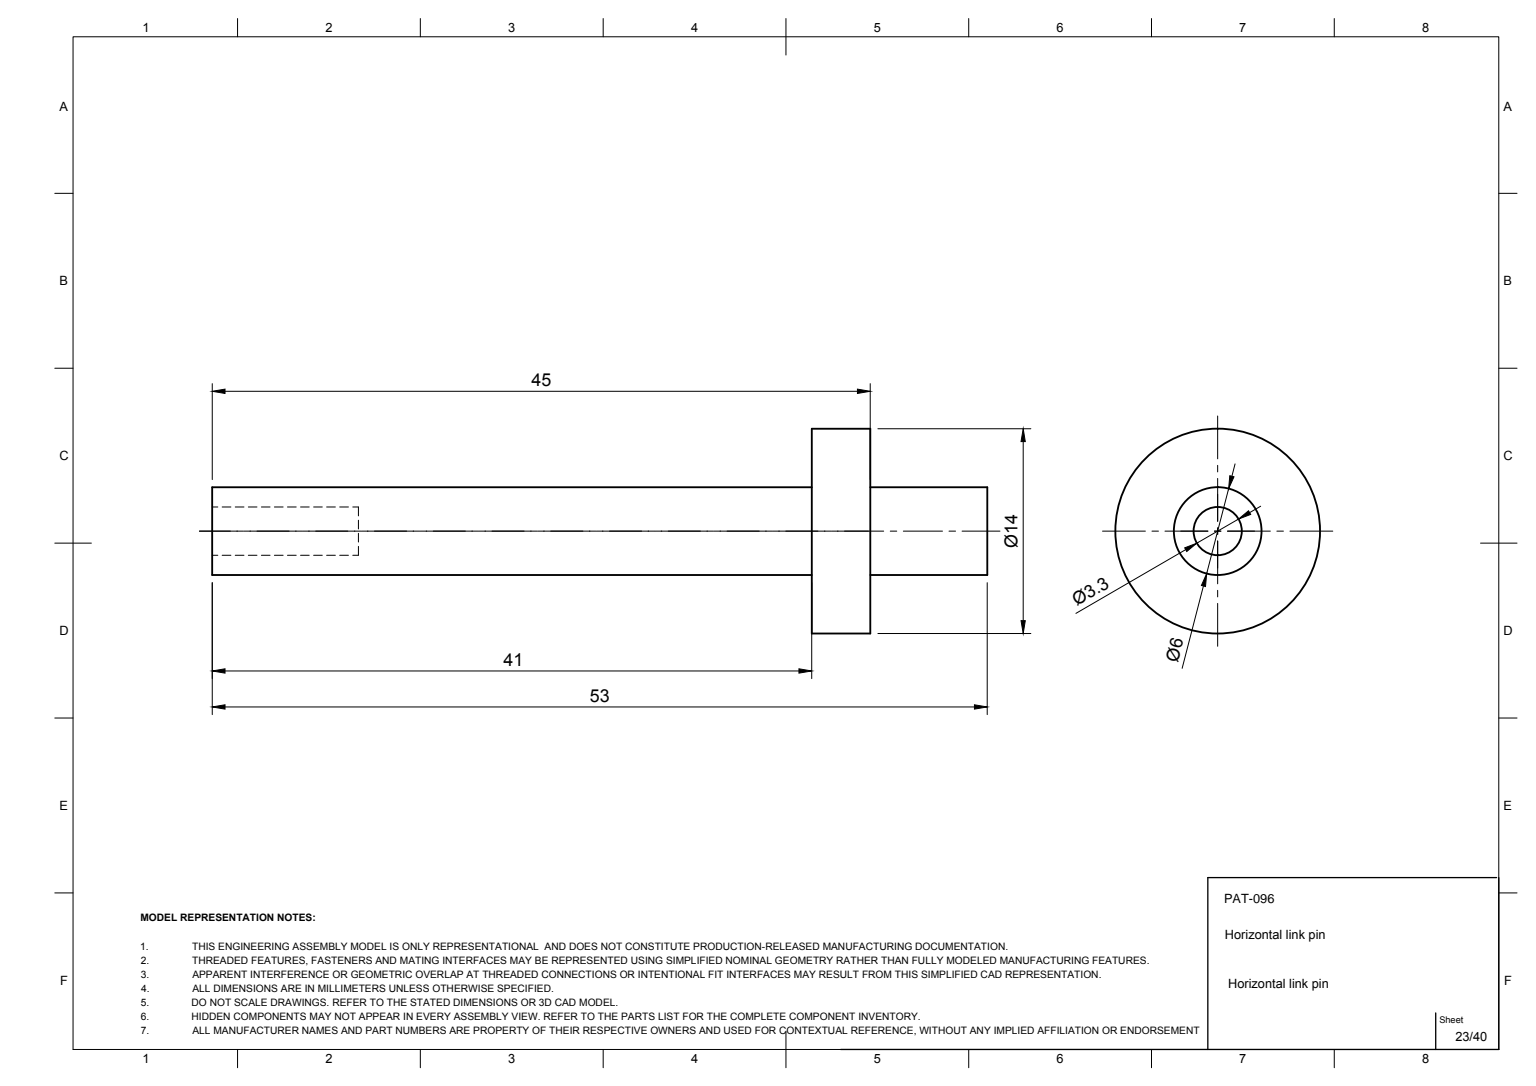
ISO-10303-21;
HEADER;
/* Generated by software containing ST-Developer
 * from STEP Tools, Inc. (www.steptools.com) 
 */

FILE_DESCRIPTION(
/* description */ ('PAT-096'),
/* implementation_level */ '2;1');

FILE_NAME(
/* name */ 'Horizontal link pin.step',
/* time_stamp */ '2026-10-29T17:03:14-07:00',
/* author */ (''),
/* organization */ (''),
/* preprocessor_version */ 'ST-DEVELOPER v20.2',
/* originating_system */ 'Autodesk Translation Framework v15.17.0.0',
/* authorisation */ '');

FILE_SCHEMA (('AUTOMOTIVE_DESIGN { 1 0 10303 214 3 1 1 }'));
ENDSEC;

DATA;
#10=MECHANICAL_DESIGN_GEOMETRIC_PRESENTATION_REPRESENTATION('',(#424),#10650);
#354=SHAPE_REPRESENTATION_RELATIONSHIP('SRR','None',#10816,#385);
#385=ADVANCED_BREP_SHAPE_REPRESENTATION('',(#461),#10634);
#424=STYLED_ITEM('',(#11064),#461);
#461=MANIFOLD_SOLID_BREP('Body1',#5559);
#559=FACE_BOUND('',#1440,.T.);
#560=FACE_BOUND('',#1442,.T.);
#561=FACE_BOUND('',#1447,.T.);
#725=PLANE('',#6395);
#726=PLANE('',#6396);
#727=PLANE('',#6399);
#728=PLANE('',#6407);
#729=PLANE('',#6408);
#1015=FACE_OUTER_BOUND('',#1437,.T.);
#1016=FACE_OUTER_BOUND('',#1438,.T.);
#1017=FACE_OUTER_BOUND('',#1439,.T.);
#1018=FACE_OUTER_BOUND('',#1441,.T.);
#1019=FACE_OUTER_BOUND('',#1443,.T.);
#1020=FACE_OUTER_BOUND('',#1444,.T.);
#1021=FACE_OUTER_BOUND('',#1445,.T.);
#1022=FACE_OUTER_BOUND('',#1446,.T.);
#1023=FACE_OUTER_BOUND('',#1448,.T.);
#1437=EDGE_LOOP('',(#4659,#4660,#4661,#4662));
#1438=EDGE_LOOP('',(#4663));
#1439=EDGE_LOOP('',(#4664));
#1440=EDGE_LOOP('',(#4665));
#1441=EDGE_LOOP('',(#4666));
#1442=EDGE_LOOP('',(#4667));
#1443=EDGE_LOOP('',(#4668,#4669,#4670,#4671));
#1444=EDGE_LOOP('',(#4672,#4673,#4674,#4675));
#1445=EDGE_LOOP('',(#4676,#4677,#4678,#4679));
#1446=EDGE_LOOP('',(#4680));
#1447=EDGE_LOOP('',(#4681));
#1448=EDGE_LOOP('',(#4682));
#1818=LINE('',#10049,#2147);
#1819=LINE('',#10063,#2148);
#1820=LINE('',#10066,#2149);
#1821=LINE('',#10071,#2150);
#2147=VECTOR('',#7846,0.165);
#2148=VECTOR('',#7865,0.7);
#2149=VECTOR('',#7868,0.3);
#2150=VECTOR('',#7875,0.3);
#2483=CIRCLE('',#6393,0.165);
#2484=CIRCLE('',#6394,0.165);
#2485=CIRCLE('',#6397,0.7);
#2486=CIRCLE('',#6398,0.3);
#2487=CIRCLE('',#6400,0.7);
#2488=CIRCLE('',#6401,0.3);
#2489=CIRCLE('',#6404,0.3);
#2490=CIRCLE('',#6406,0.3);
#2899=VERTEX_POINT('',#10046);
#2900=VERTEX_POINT('',#10048);
#2901=VERTEX_POINT('',#10053);
#2902=VERTEX_POINT('',#10055);
#2903=VERTEX_POINT('',#10058);
#2904=VERTEX_POINT('',#10060);
#2905=VERTEX_POINT('',#10065);
#2906=VERTEX_POINT('',#10069);
#3508=EDGE_CURVE('',#2899,#2899,#2483,.T.);
#3509=EDGE_CURVE('',#2899,#2900,#1818,.T.);
#3510=EDGE_CURVE('',#2900,#2900,#2484,.T.);
#3511=EDGE_CURVE('',#2901,#2901,#2485,.T.);
#3512=EDGE_CURVE('',#2902,#2902,#2486,.T.);
#3513=EDGE_CURVE('',#2903,#2903,#2487,.T.);
#3514=EDGE_CURVE('',#2904,#2904,#2488,.T.);
#3515=EDGE_CURVE('',#2901,#2903,#1819,.T.);
#3516=EDGE_CURVE('',#2904,#2905,#1820,.T.);
#3517=EDGE_CURVE('',#2905,#2905,#2489,.T.);
#3518=EDGE_CURVE('',#2906,#2906,#2490,.T.);
#3519=EDGE_CURVE('',#2906,#2902,#1821,.T.);
#4659=ORIENTED_EDGE('',*,*,#3508,.F.);
#4660=ORIENTED_EDGE('',*,*,#3509,.T.);
#4661=ORIENTED_EDGE('',*,*,#3510,.F.);
#4662=ORIENTED_EDGE('',*,*,#3509,.F.);
#4663=ORIENTED_EDGE('',*,*,#3508,.T.);
#4664=ORIENTED_EDGE('',*,*,#3511,.T.);
#4665=ORIENTED_EDGE('',*,*,#3512,.F.);
#4666=ORIENTED_EDGE('',*,*,#3513,.F.);
#4667=ORIENTED_EDGE('',*,*,#3514,.F.);
#4668=ORIENTED_EDGE('',*,*,#3511,.F.);
#4669=ORIENTED_EDGE('',*,*,#3515,.T.);
#4670=ORIENTED_EDGE('',*,*,#3513,.T.);
#4671=ORIENTED_EDGE('',*,*,#3515,.F.);
#4672=ORIENTED_EDGE('',*,*,#3514,.T.);
#4673=ORIENTED_EDGE('',*,*,#3516,.T.);
#4674=ORIENTED_EDGE('',*,*,#3517,.T.);
#4675=ORIENTED_EDGE('',*,*,#3516,.F.);
#4676=ORIENTED_EDGE('',*,*,#3518,.F.);
#4677=ORIENTED_EDGE('',*,*,#3519,.T.);
#4678=ORIENTED_EDGE('',*,*,#3512,.T.);
#4679=ORIENTED_EDGE('',*,*,#3519,.F.);
#4680=ORIENTED_EDGE('',*,*,#3518,.T.);
#4681=ORIENTED_EDGE('',*,*,#3510,.T.);
#4682=ORIENTED_EDGE('',*,*,#3517,.F.);
#5152=CYLINDRICAL_SURFACE('',#6392,0.165);
#5153=CYLINDRICAL_SURFACE('',#6402,0.7);
#5154=CYLINDRICAL_SURFACE('',#6403,0.3);
#5155=CYLINDRICAL_SURFACE('',#6405,0.3);
#5420=ADVANCED_FACE('',(#1015),#5152,.F.);
#5421=ADVANCED_FACE('',(#1016),#725,.T.);
#5422=ADVANCED_FACE('',(#1017,#559),#726,.T.);
#5423=ADVANCED_FACE('',(#1018,#560),#727,.F.);
#5424=ADVANCED_FACE('',(#1019),#5153,.T.);
#5425=ADVANCED_FACE('',(#1020),#5154,.T.);
#5426=ADVANCED_FACE('',(#1021),#5155,.T.);
#5427=ADVANCED_FACE('',(#1022,#561),#728,.T.);
#5428=ADVANCED_FACE('',(#1023),#729,.F.);
#5559=CLOSED_SHELL('',(#5420,#5421,#5422,#5423,#5424,#5425,#5426,#5427,
#5428));
#6391=AXIS2_PLACEMENT_3D('',#10044,#7840,#7841);
#6392=AXIS2_PLACEMENT_3D('',#10045,#7842,#7843);
#6393=AXIS2_PLACEMENT_3D('',#10047,#7844,#7845);
#6394=AXIS2_PLACEMENT_3D('',#10050,#7847,#7848);
#6395=AXIS2_PLACEMENT_3D('',#10051,#7849,#7850);
#6396=AXIS2_PLACEMENT_3D('',#10052,#7851,#7852);
#6397=AXIS2_PLACEMENT_3D('',#10054,#7853,#7854);
#6398=AXIS2_PLACEMENT_3D('',#10056,#7855,#7856);
#6399=AXIS2_PLACEMENT_3D('',#10057,#7857,#7858);
#6400=AXIS2_PLACEMENT_3D('',#10059,#7859,#7860);
#6401=AXIS2_PLACEMENT_3D('',#10061,#7861,#7862);
#6402=AXIS2_PLACEMENT_3D('',#10062,#7863,#7864);
#6403=AXIS2_PLACEMENT_3D('',#10064,#7866,#7867);
#6404=AXIS2_PLACEMENT_3D('',#10067,#7869,#7870);
#6405=AXIS2_PLACEMENT_3D('',#10068,#7871,#7872);
#6406=AXIS2_PLACEMENT_3D('',#10070,#7873,#7874);
#6407=AXIS2_PLACEMENT_3D('',#10072,#7876,#7877);
#6408=AXIS2_PLACEMENT_3D('',#10073,#7878,#7879);
#7840=DIRECTION('axis',(0.,0.,1.));
#7841=DIRECTION('refdir',(1.,0.,0.));
#7842=DIRECTION('center_axis',(0.,0.,1.));
#7843=DIRECTION('ref_axis',(1.,0.,0.));
#7844=DIRECTION('center_axis',(0.,0.,1.));
#7845=DIRECTION('ref_axis',(1.,0.,0.));
#7846=DIRECTION('',(0.,0.,1.));
#7847=DIRECTION('center_axis',(0.,0.,-1.));
#7848=DIRECTION('ref_axis',(1.,0.,0.));
#7849=DIRECTION('center_axis',(0.,0.,1.));
#7850=DIRECTION('ref_axis',(1.,0.,0.));
#7851=DIRECTION('center_axis',(0.,0.,1.));
#7852=DIRECTION('ref_axis',(1.,0.,0.));
#7853=DIRECTION('center_axis',(0.,0.,1.));
#7854=DIRECTION('ref_axis',(1.,0.,0.));
#7855=DIRECTION('center_axis',(0.,0.,1.));
#7856=DIRECTION('ref_axis',(1.,0.,0.));
#7857=DIRECTION('center_axis',(0.,0.,1.));
#7858=DIRECTION('ref_axis',(1.,0.,0.));
#7859=DIRECTION('center_axis',(0.,0.,1.));
#7860=DIRECTION('ref_axis',(1.,0.,0.));
#7861=DIRECTION('center_axis',(0.,0.,-1.));
#7862=DIRECTION('ref_axis',(1.,0.,0.));
#7863=DIRECTION('center_axis',(0.,0.,1.));
#7864=DIRECTION('ref_axis',(1.,0.,0.));
#7865=DIRECTION('',(0.,0.,-1.));
#7866=DIRECTION('center_axis',(0.,0.,1.));
#7867=DIRECTION('ref_axis',(1.,0.,0.));
#7868=DIRECTION('',(0.,0.,-1.));
#7869=DIRECTION('center_axis',(0.,0.,1.));
#7870=DIRECTION('ref_axis',(1.,0.,0.));
#7871=DIRECTION('center_axis',(0.,0.,1.));
#7872=DIRECTION('ref_axis',(1.,0.,0.));
#7873=DIRECTION('center_axis',(0.,0.,1.));
#7874=DIRECTION('ref_axis',(1.,0.,0.));
#7875=DIRECTION('',(0.,0.,-1.));
#7876=DIRECTION('center_axis',(0.,0.,1.));
#7877=DIRECTION('ref_axis',(1.,0.,0.));
#7878=DIRECTION('center_axis',(0.,0.,1.));
#7879=DIRECTION('ref_axis',(1.,0.,0.));
#10044=CARTESIAN_POINT('',(0.,0.,0.));
#10045=CARTESIAN_POINT('Origin',(0.,2.,9.1));
#10046=CARTESIAN_POINT('',(-0.165,2.,9.1));
#10047=CARTESIAN_POINT('Origin',(0.,2.,9.1));
#10048=CARTESIAN_POINT('',(-0.165,2.,10.1));
#10049=CARTESIAN_POINT('',(-0.165,2.,9.1));
#10050=CARTESIAN_POINT('Origin',(0.,2.,10.1));
#10051=CARTESIAN_POINT('Origin',(0.,2.,9.1));
#10052=CARTESIAN_POINT('Origin',(0.,2.,6.));
#10053=CARTESIAN_POINT('',(-0.7,2.,6.));
#10054=CARTESIAN_POINT('Origin',(0.,2.,6.));
#10055=CARTESIAN_POINT('',(-0.3,2.,6.));
#10056=CARTESIAN_POINT('Origin',(0.,2.,6.));
#10057=CARTESIAN_POINT('Origin',(0.,2.,5.6));
#10058=CARTESIAN_POINT('',(-0.7,2.,5.6));
#10059=CARTESIAN_POINT('Origin',(0.,2.,5.6));
#10060=CARTESIAN_POINT('',(-0.3,2.,5.6));
#10061=CARTESIAN_POINT('Origin',(0.,2.,5.6));
#10062=CARTESIAN_POINT('Origin',(0.,2.,5.6));
#10063=CARTESIAN_POINT('',(-0.7,2.,5.6));
#10064=CARTESIAN_POINT('Origin',(0.,2.,4.8));
#10065=CARTESIAN_POINT('',(-0.3,2.,4.8));
#10066=CARTESIAN_POINT('',(-0.3,2.,4.8));
#10067=CARTESIAN_POINT('Origin',(0.,2.,4.8));
#10068=CARTESIAN_POINT('Origin',(0.,2.,4.8));
#10069=CARTESIAN_POINT('',(-0.3,2.,10.1));
#10070=CARTESIAN_POINT('Origin',(0.,2.,10.1));
#10071=CARTESIAN_POINT('',(-0.3,2.,4.8));
#10072=CARTESIAN_POINT('Origin',(0.,2.,10.1));
#10073=CARTESIAN_POINT('Origin',(0.,2.,4.8));
#10595=UNCERTAINTY_MEASURE_WITH_UNIT(LENGTH_MEASURE(0.001),#10651,
'DISTANCE_ACCURACY_VALUE',
'Maximum model space distance between geometric entities at asserted c
onnectivities');
#10611=UNCERTAINTY_MEASURE_WITH_UNIT(LENGTH_MEASURE(0.001),#10651,
'DISTANCE_ACCURACY_VALUE',
'Maximum model space distance between geometric entities at asserted c
onnectivities');
#10634=(
GEOMETRIC_REPRESENTATION_CONTEXT(3)
GLOBAL_UNCERTAINTY_ASSIGNED_CONTEXT((#10595))
GLOBAL_UNIT_ASSIGNED_CONTEXT((#10651,#10653,#10654))
REPRESENTATION_CONTEXT('','3D')
);
#10650=(
GEOMETRIC_REPRESENTATION_CONTEXT(3)
GLOBAL_UNCERTAINTY_ASSIGNED_CONTEXT((#10611))
GLOBAL_UNIT_ASSIGNED_CONTEXT((#10651,#10653,#10654))
REPRESENTATION_CONTEXT('','3D')
);
#10651=(
LENGTH_UNIT()
NAMED_UNIT(*)
SI_UNIT(.CENTI.,.METRE.)
);
#10653=(
NAMED_UNIT(*)
PLANE_ANGLE_UNIT()
SI_UNIT($,.RADIAN.)
);
#10654=(
NAMED_UNIT(*)
SI_UNIT($,.STERADIAN.)
SOLID_ANGLE_UNIT()
);
#10677=SHAPE_DEFINITION_REPRESENTATION(#10720,#10816);
#10720=PRODUCT_DEFINITION_SHAPE('',$,#10855);
#10816=SHAPE_REPRESENTATION('',(#6391),#10634);
#10832=PRODUCT_DEFINITION_CONTEXT('part definition',#10948,'design');
#10855=PRODUCT_DEFINITION('Horizontal link pin','Horizontal link pin',#10893,
#10832);
#10893=PRODUCT_DEFINITION_FORMATION('',$,#10972);
#10948=APPLICATION_CONTEXT(
'Core Data for Automotive Mechanical Design Process');
#10949=PRODUCT_CONTEXT('part definition',#10948,'mechanical');
#10972=PRODUCT('Horizontal link pin','Horizontal link pin',
'Horizontal link pin',(#10949));
#11058=COLOUR_RGB('Grey',0.48,0.52,0.57);
#11059=FILL_AREA_STYLE_COLOUR('',#11058);
#11060=FILL_AREA_STYLE('',(#11059));
#11061=SURFACE_STYLE_FILL_AREA(#11060);
#11062=SURFACE_SIDE_STYLE('',(#11061));
#11063=SURFACE_STYLE_USAGE(.BOTH.,#11062);
#11064=PRESENTATION_STYLE_ASSIGNMENT((#11063));
ENDSEC;
END-ISO-10303-21;
